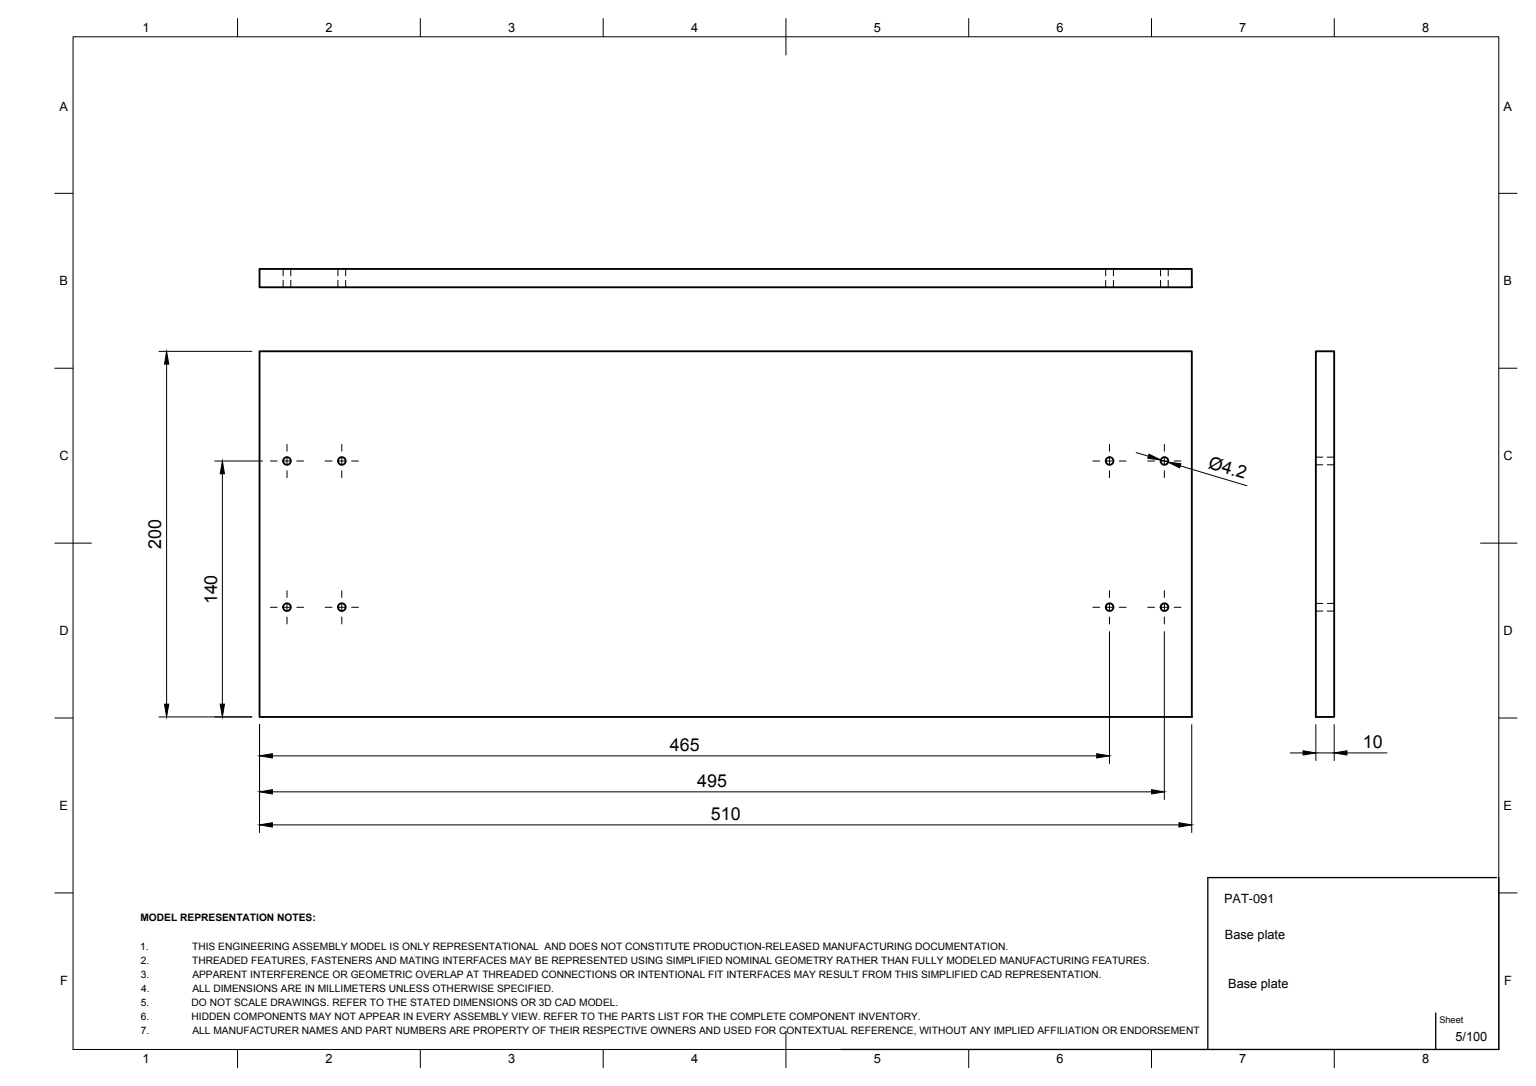
ISO-10303-21;
HEADER;
/* Generated by software containing ST-Developer
 * from STEP Tools, Inc. (www.steptools.com) 
 */

FILE_DESCRIPTION(
/* description */ ('PAT-091'),
/* implementation_level */ '2;1');

FILE_NAME(
/* name */ 'Base plate.step',
/* time_stamp */ '2026-10-27T15:34:44-07:00',
/* author */ (''),
/* organization */ (''),
/* preprocessor_version */ 'ST-DEVELOPER v20.2',
/* originating_system */ 'Autodesk Translation Framework v15.17.0.0',
/* authorisation */ '');

FILE_SCHEMA (('AUTOMOTIVE_DESIGN { 1 0 10303 214 3 1 1 }'));
ENDSEC;

DATA;
#10=MECHANICAL_DESIGN_GEOMETRIC_PRESENTATION_REPRESENTATION('',(#971),#25100);
#751=SHAPE_REPRESENTATION_RELATIONSHIP('SRR','None',#25512,#861);
#861=ADVANCED_BREP_SHAPE_REPRESENTATION('',(#1095),#24982);
#971=STYLED_ITEM('',(#26170),#1095);
#1095=MANIFOLD_SOLID_BREP('Body1',#13248);
#1215=FACE_BOUND('',#2894,.T.);
#1216=FACE_BOUND('',#2895,.T.);
#1217=FACE_BOUND('',#2896,.T.);
#1218=FACE_BOUND('',#2897,.T.);
#1219=FACE_BOUND('',#2898,.T.);
#1220=FACE_BOUND('',#2899,.T.);
#1221=FACE_BOUND('',#2900,.T.);
#1222=FACE_BOUND('',#2901,.T.);
#1223=FACE_BOUND('',#2903,.T.);
#1224=FACE_BOUND('',#2904,.T.);
#1225=FACE_BOUND('',#2905,.T.);
#1226=FACE_BOUND('',#2906,.T.);
#1227=FACE_BOUND('',#2907,.T.);
#1228=FACE_BOUND('',#2908,.T.);
#1229=FACE_BOUND('',#2909,.T.);
#1230=FACE_BOUND('',#2910,.T.);
#1640=PLANE('',#14612);
#1641=PLANE('',#14613);
#1642=PLANE('',#14614);
#1643=PLANE('',#14615);
#1644=PLANE('',#14616);
#1645=PLANE('',#14617);
#2063=FACE_OUTER_BOUND('',#2881,.T.);
#2064=FACE_OUTER_BOUND('',#2882,.T.);
#2065=FACE_OUTER_BOUND('',#2883,.T.);
#2066=FACE_OUTER_BOUND('',#2884,.T.);
#2067=FACE_OUTER_BOUND('',#2885,.T.);
#2068=FACE_OUTER_BOUND('',#2886,.T.);
#2069=FACE_OUTER_BOUND('',#2887,.T.);
#2070=FACE_OUTER_BOUND('',#2888,.T.);
#2071=FACE_OUTER_BOUND('',#2889,.T.);
#2072=FACE_OUTER_BOUND('',#2890,.T.);
#2073=FACE_OUTER_BOUND('',#2891,.T.);
#2074=FACE_OUTER_BOUND('',#2892,.T.);
#2075=FACE_OUTER_BOUND('',#2893,.T.);
#2076=FACE_OUTER_BOUND('',#2902,.T.);
#2881=EDGE_LOOP('',(#8972,#8973,#8974,#8975));
#2882=EDGE_LOOP('',(#8976,#8977,#8978,#8979));
#2883=EDGE_LOOP('',(#8980,#8981,#8982,#8983));
#2884=EDGE_LOOP('',(#8984,#8985,#8986,#8987));
#2885=EDGE_LOOP('',(#8988,#8989,#8990,#8991));
#2886=EDGE_LOOP('',(#8992,#8993,#8994,#8995));
#2887=EDGE_LOOP('',(#8996,#8997,#8998,#8999));
#2888=EDGE_LOOP('',(#9000,#9001,#9002,#9003));
#2889=EDGE_LOOP('',(#9004,#9005,#9006,#9007));
#2890=EDGE_LOOP('',(#9008,#9009,#9010,#9011));
#2891=EDGE_LOOP('',(#9012,#9013,#9014,#9015));
#2892=EDGE_LOOP('',(#9016,#9017,#9018,#9019));
#2893=EDGE_LOOP('',(#9020,#9021,#9022,#9023));
#2894=EDGE_LOOP('',(#9024));
#2895=EDGE_LOOP('',(#9025));
#2896=EDGE_LOOP('',(#9026));
#2897=EDGE_LOOP('',(#9027));
#2898=EDGE_LOOP('',(#9028));
#2899=EDGE_LOOP('',(#9029));
#2900=EDGE_LOOP('',(#9030));
#2901=EDGE_LOOP('',(#9031));
#2902=EDGE_LOOP('',(#9032,#9033,#9034,#9035));
#2903=EDGE_LOOP('',(#9036));
#2904=EDGE_LOOP('',(#9037));
#2905=EDGE_LOOP('',(#9038));
#2906=EDGE_LOOP('',(#9039));
#2907=EDGE_LOOP('',(#9040));
#2908=EDGE_LOOP('',(#9041));
#2909=EDGE_LOOP('',(#9042));
#2910=EDGE_LOOP('',(#9043));
#4124=LINE('',#20981,#4864);
#4125=LINE('',#20987,#4865);
#4126=LINE('',#20993,#4866);
#4127=LINE('',#20999,#4867);
#4128=LINE('',#21005,#4868);
#4129=LINE('',#21011,#4869);
#4130=LINE('',#21017,#4870);
#4131=LINE('',#21023,#4871);
#4132=LINE('',#21028,#4872);
#4133=LINE('',#21030,#4873);
#4134=LINE('',#21032,#4874);
#4135=LINE('',#21033,#4875);
#4136=LINE('',#21036,#4876);
#4137=LINE('',#21038,#4877);
#4138=LINE('',#21039,#4878);
#4139=LINE('',#21042,#4879);
#4140=LINE('',#21044,#4880);
#4141=LINE('',#21045,#4881);
#4142=LINE('',#21047,#4882);
#4143=LINE('',#21048,#4883);
#4864=VECTOR('',#16478,0.210000000000001);
#4865=VECTOR('',#16485,0.210000000000001);
#4866=VECTOR('',#16492,0.210000000000001);
#4867=VECTOR('',#16499,0.210000000000001);
#4868=VECTOR('',#16506,0.21);
#4869=VECTOR('',#16513,0.21);
#4870=VECTOR('',#16520,0.21);
#4871=VECTOR('',#16527,0.21);
#4872=VECTOR('',#16532,1.);
#4873=VECTOR('',#16533,1.);
#4874=VECTOR('',#16534,1.);
#4875=VECTOR('',#16535,1.);
#4876=VECTOR('',#16538,1.);
#4877=VECTOR('',#16539,1.);
#4878=VECTOR('',#16540,1.);
#4879=VECTOR('',#16543,1.);
#4880=VECTOR('',#16544,1.);
#4881=VECTOR('',#16545,1.);
#4882=VECTOR('',#16548,1.);
#4883=VECTOR('',#16549,1.);
#5604=CIRCLE('',#14589,0.210000000000001);
#5605=CIRCLE('',#14590,0.210000000000001);
#5606=CIRCLE('',#14592,0.210000000000001);
#5607=CIRCLE('',#14593,0.210000000000001);
#5608=CIRCLE('',#14595,0.210000000000001);
#5609=CIRCLE('',#14596,0.210000000000001);
#5610=CIRCLE('',#14598,0.210000000000001);
#5611=CIRCLE('',#14599,0.210000000000001);
#5612=CIRCLE('',#14601,0.21);
#5613=CIRCLE('',#14602,0.21);
#5614=CIRCLE('',#14604,0.21);
#5615=CIRCLE('',#14605,0.21);
#5616=CIRCLE('',#14607,0.21);
#5617=CIRCLE('',#14608,0.21);
#5618=CIRCLE('',#14610,0.21);
#5619=CIRCLE('',#14611,0.21);
#6383=VERTEX_POINT('',#20978);
#6384=VERTEX_POINT('',#20980);
#6385=VERTEX_POINT('',#20984);
#6386=VERTEX_POINT('',#20986);
#6387=VERTEX_POINT('',#20990);
#6388=VERTEX_POINT('',#20992);
#6389=VERTEX_POINT('',#20996);
#6390=VERTEX_POINT('',#20998);
#6391=VERTEX_POINT('',#21002);
#6392=VERTEX_POINT('',#21004);
#6393=VERTEX_POINT('',#21008);
#6394=VERTEX_POINT('',#21010);
#6395=VERTEX_POINT('',#21014);
#6396=VERTEX_POINT('',#21016);
#6397=VERTEX_POINT('',#21020);
#6398=VERTEX_POINT('',#21022);
#6399=VERTEX_POINT('',#21026);
#6400=VERTEX_POINT('',#21027);
#6401=VERTEX_POINT('',#21029);
#6402=VERTEX_POINT('',#21031);
#6403=VERTEX_POINT('',#21035);
#6404=VERTEX_POINT('',#21037);
#6405=VERTEX_POINT('',#21041);
#6406=VERTEX_POINT('',#21043);
#7421=EDGE_CURVE('',#6383,#6383,#5604,.T.);
#7422=EDGE_CURVE('',#6383,#6384,#4124,.T.);
#7423=EDGE_CURVE('',#6384,#6384,#5605,.T.);
#7424=EDGE_CURVE('',#6385,#6385,#5606,.T.);
#7425=EDGE_CURVE('',#6385,#6386,#4125,.T.);
#7426=EDGE_CURVE('',#6386,#6386,#5607,.T.);
#7427=EDGE_CURVE('',#6387,#6387,#5608,.T.);
#7428=EDGE_CURVE('',#6387,#6388,#4126,.T.);
#7429=EDGE_CURVE('',#6388,#6388,#5609,.T.);
#7430=EDGE_CURVE('',#6389,#6389,#5610,.T.);
#7431=EDGE_CURVE('',#6389,#6390,#4127,.T.);
#7432=EDGE_CURVE('',#6390,#6390,#5611,.T.);
#7433=EDGE_CURVE('',#6391,#6391,#5612,.T.);
#7434=EDGE_CURVE('',#6391,#6392,#4128,.T.);
#7435=EDGE_CURVE('',#6392,#6392,#5613,.T.);
#7436=EDGE_CURVE('',#6393,#6393,#5614,.T.);
#7437=EDGE_CURVE('',#6393,#6394,#4129,.T.);
#7438=EDGE_CURVE('',#6394,#6394,#5615,.T.);
#7439=EDGE_CURVE('',#6395,#6395,#5616,.T.);
#7440=EDGE_CURVE('',#6395,#6396,#4130,.T.);
#7441=EDGE_CURVE('',#6396,#6396,#5617,.T.);
#7442=EDGE_CURVE('',#6397,#6397,#5618,.T.);
#7443=EDGE_CURVE('',#6397,#6398,#4131,.T.);
#7444=EDGE_CURVE('',#6398,#6398,#5619,.T.);
#7445=EDGE_CURVE('',#6399,#6400,#4132,.T.);
#7446=EDGE_CURVE('',#6400,#6401,#4133,.T.);
#7447=EDGE_CURVE('',#6402,#6401,#4134,.T.);
#7448=EDGE_CURVE('',#6399,#6402,#4135,.T.);
#7449=EDGE_CURVE('',#6403,#6399,#4136,.T.);
#7450=EDGE_CURVE('',#6404,#6402,#4137,.T.);
#7451=EDGE_CURVE('',#6403,#6404,#4138,.T.);
#7452=EDGE_CURVE('',#6405,#6403,#4139,.T.);
#7453=EDGE_CURVE('',#6406,#6404,#4140,.T.);
#7454=EDGE_CURVE('',#6405,#6406,#4141,.T.);
#7455=EDGE_CURVE('',#6400,#6405,#4142,.T.);
#7456=EDGE_CURVE('',#6401,#6406,#4143,.T.);
#8972=ORIENTED_EDGE('',*,*,#7421,.F.);
#8973=ORIENTED_EDGE('',*,*,#7422,.T.);
#8974=ORIENTED_EDGE('',*,*,#7423,.F.);
#8975=ORIENTED_EDGE('',*,*,#7422,.F.);
#8976=ORIENTED_EDGE('',*,*,#7424,.F.);
#8977=ORIENTED_EDGE('',*,*,#7425,.T.);
#8978=ORIENTED_EDGE('',*,*,#7426,.F.);
#8979=ORIENTED_EDGE('',*,*,#7425,.F.);
#8980=ORIENTED_EDGE('',*,*,#7427,.F.);
#8981=ORIENTED_EDGE('',*,*,#7428,.T.);
#8982=ORIENTED_EDGE('',*,*,#7429,.F.);
#8983=ORIENTED_EDGE('',*,*,#7428,.F.);
#8984=ORIENTED_EDGE('',*,*,#7430,.F.);
#8985=ORIENTED_EDGE('',*,*,#7431,.T.);
#8986=ORIENTED_EDGE('',*,*,#7432,.F.);
#8987=ORIENTED_EDGE('',*,*,#7431,.F.);
#8988=ORIENTED_EDGE('',*,*,#7433,.F.);
#8989=ORIENTED_EDGE('',*,*,#7434,.T.);
#8990=ORIENTED_EDGE('',*,*,#7435,.F.);
#8991=ORIENTED_EDGE('',*,*,#7434,.F.);
#8992=ORIENTED_EDGE('',*,*,#7436,.F.);
#8993=ORIENTED_EDGE('',*,*,#7437,.T.);
#8994=ORIENTED_EDGE('',*,*,#7438,.F.);
#8995=ORIENTED_EDGE('',*,*,#7437,.F.);
#8996=ORIENTED_EDGE('',*,*,#7439,.F.);
#8997=ORIENTED_EDGE('',*,*,#7440,.T.);
#8998=ORIENTED_EDGE('',*,*,#7441,.F.);
#8999=ORIENTED_EDGE('',*,*,#7440,.F.);
#9000=ORIENTED_EDGE('',*,*,#7442,.F.);
#9001=ORIENTED_EDGE('',*,*,#7443,.T.);
#9002=ORIENTED_EDGE('',*,*,#7444,.F.);
#9003=ORIENTED_EDGE('',*,*,#7443,.F.);
#9004=ORIENTED_EDGE('',*,*,#7445,.T.);
#9005=ORIENTED_EDGE('',*,*,#7446,.T.);
#9006=ORIENTED_EDGE('',*,*,#7447,.F.);
#9007=ORIENTED_EDGE('',*,*,#7448,.F.);
#9008=ORIENTED_EDGE('',*,*,#7449,.T.);
#9009=ORIENTED_EDGE('',*,*,#7448,.T.);
#9010=ORIENTED_EDGE('',*,*,#7450,.F.);
#9011=ORIENTED_EDGE('',*,*,#7451,.F.);
#9012=ORIENTED_EDGE('',*,*,#7452,.T.);
#9013=ORIENTED_EDGE('',*,*,#7451,.T.);
#9014=ORIENTED_EDGE('',*,*,#7453,.F.);
#9015=ORIENTED_EDGE('',*,*,#7454,.F.);
#9016=ORIENTED_EDGE('',*,*,#7455,.T.);
#9017=ORIENTED_EDGE('',*,*,#7454,.T.);
#9018=ORIENTED_EDGE('',*,*,#7456,.F.);
#9019=ORIENTED_EDGE('',*,*,#7446,.F.);
#9020=ORIENTED_EDGE('',*,*,#7456,.T.);
#9021=ORIENTED_EDGE('',*,*,#7453,.T.);
#9022=ORIENTED_EDGE('',*,*,#7450,.T.);
#9023=ORIENTED_EDGE('',*,*,#7447,.T.);
#9024=ORIENTED_EDGE('',*,*,#7444,.T.);
#9025=ORIENTED_EDGE('',*,*,#7441,.T.);
#9026=ORIENTED_EDGE('',*,*,#7438,.T.);
#9027=ORIENTED_EDGE('',*,*,#7435,.T.);
#9028=ORIENTED_EDGE('',*,*,#7432,.T.);
#9029=ORIENTED_EDGE('',*,*,#7429,.T.);
#9030=ORIENTED_EDGE('',*,*,#7426,.T.);
#9031=ORIENTED_EDGE('',*,*,#7423,.T.);
#9032=ORIENTED_EDGE('',*,*,#7455,.F.);
#9033=ORIENTED_EDGE('',*,*,#7445,.F.);
#9034=ORIENTED_EDGE('',*,*,#7449,.F.);
#9035=ORIENTED_EDGE('',*,*,#7452,.F.);
#9036=ORIENTED_EDGE('',*,*,#7442,.T.);
#9037=ORIENTED_EDGE('',*,*,#7439,.T.);
#9038=ORIENTED_EDGE('',*,*,#7436,.T.);
#9039=ORIENTED_EDGE('',*,*,#7433,.T.);
#9040=ORIENTED_EDGE('',*,*,#7430,.T.);
#9041=ORIENTED_EDGE('',*,*,#7427,.T.);
#9042=ORIENTED_EDGE('',*,*,#7424,.T.);
#9043=ORIENTED_EDGE('',*,*,#7421,.T.);
#12074=CYLINDRICAL_SURFACE('',#14588,0.210000000000001);
#12075=CYLINDRICAL_SURFACE('',#14591,0.210000000000001);
#12076=CYLINDRICAL_SURFACE('',#14594,0.210000000000001);
#12077=CYLINDRICAL_SURFACE('',#14597,0.210000000000001);
#12078=CYLINDRICAL_SURFACE('',#14600,0.21);
#12079=CYLINDRICAL_SURFACE('',#14603,0.21);
#12080=CYLINDRICAL_SURFACE('',#14606,0.21);
#12081=CYLINDRICAL_SURFACE('',#14609,0.21);
#12430=ADVANCED_FACE('',(#2063),#12074,.F.);
#12431=ADVANCED_FACE('',(#2064),#12075,.F.);
#12432=ADVANCED_FACE('',(#2065),#12076,.F.);
#12433=ADVANCED_FACE('',(#2066),#12077,.F.);
#12434=ADVANCED_FACE('',(#2067),#12078,.F.);
#12435=ADVANCED_FACE('',(#2068),#12079,.F.);
#12436=ADVANCED_FACE('',(#2069),#12080,.F.);
#12437=ADVANCED_FACE('',(#2070),#12081,.F.);
#12438=ADVANCED_FACE('',(#2071),#1640,.T.);
#12439=ADVANCED_FACE('',(#2072),#1641,.T.);
#12440=ADVANCED_FACE('',(#2073),#1642,.T.);
#12441=ADVANCED_FACE('',(#2074),#1643,.T.);
#12442=ADVANCED_FACE('',(#2075,#1215,#1216,#1217,#1218,#1219,#1220,#1221,
#1222),#1644,.T.);
#12443=ADVANCED_FACE('',(#2076,#1223,#1224,#1225,#1226,#1227,#1228,#1229,
#1230),#1645,.F.);
#13248=CLOSED_SHELL('',(#12430,#12431,#12432,#12433,#12434,#12435,#12436,
#12437,#12438,#12439,#12440,#12441,#12442,#12443));
#14587=AXIS2_PLACEMENT_3D('',#20976,#16472,#16473);
#14588=AXIS2_PLACEMENT_3D('',#20977,#16474,#16475);
#14589=AXIS2_PLACEMENT_3D('',#20979,#16476,#16477);
#14590=AXIS2_PLACEMENT_3D('',#20982,#16479,#16480);
#14591=AXIS2_PLACEMENT_3D('',#20983,#16481,#16482);
#14592=AXIS2_PLACEMENT_3D('',#20985,#16483,#16484);
#14593=AXIS2_PLACEMENT_3D('',#20988,#16486,#16487);
#14594=AXIS2_PLACEMENT_3D('',#20989,#16488,#16489);
#14595=AXIS2_PLACEMENT_3D('',#20991,#16490,#16491);
#14596=AXIS2_PLACEMENT_3D('',#20994,#16493,#16494);
#14597=AXIS2_PLACEMENT_3D('',#20995,#16495,#16496);
#14598=AXIS2_PLACEMENT_3D('',#20997,#16497,#16498);
#14599=AXIS2_PLACEMENT_3D('',#21000,#16500,#16501);
#14600=AXIS2_PLACEMENT_3D('',#21001,#16502,#16503);
#14601=AXIS2_PLACEMENT_3D('',#21003,#16504,#16505);
#14602=AXIS2_PLACEMENT_3D('',#21006,#16507,#16508);
#14603=AXIS2_PLACEMENT_3D('',#21007,#16509,#16510);
#14604=AXIS2_PLACEMENT_3D('',#21009,#16511,#16512);
#14605=AXIS2_PLACEMENT_3D('',#21012,#16514,#16515);
#14606=AXIS2_PLACEMENT_3D('',#21013,#16516,#16517);
#14607=AXIS2_PLACEMENT_3D('',#21015,#16518,#16519);
#14608=AXIS2_PLACEMENT_3D('',#21018,#16521,#16522);
#14609=AXIS2_PLACEMENT_3D('',#21019,#16523,#16524);
#14610=AXIS2_PLACEMENT_3D('',#21021,#16525,#16526);
#14611=AXIS2_PLACEMENT_3D('',#21024,#16528,#16529);
#14612=AXIS2_PLACEMENT_3D('',#21025,#16530,#16531);
#14613=AXIS2_PLACEMENT_3D('',#21034,#16536,#16537);
#14614=AXIS2_PLACEMENT_3D('',#21040,#16541,#16542);
#14615=AXIS2_PLACEMENT_3D('',#21046,#16546,#16547);
#14616=AXIS2_PLACEMENT_3D('',#21049,#16550,#16551);
#14617=AXIS2_PLACEMENT_3D('',#21050,#16552,#16553);
#16472=DIRECTION('axis',(0.,0.,1.));
#16473=DIRECTION('refdir',(1.,0.,0.));
#16474=DIRECTION('center_axis',(0.,0.,1.));
#16475=DIRECTION('ref_axis',(1.,0.,0.));
#16476=DIRECTION('center_axis',(0.,0.,1.));
#16477=DIRECTION('ref_axis',(1.,0.,0.));
#16478=DIRECTION('',(0.,0.,1.));
#16479=DIRECTION('center_axis',(0.,0.,-1.));
#16480=DIRECTION('ref_axis',(1.,0.,0.));
#16481=DIRECTION('center_axis',(0.,0.,1.));
#16482=DIRECTION('ref_axis',(1.,0.,0.));
#16483=DIRECTION('center_axis',(0.,0.,1.));
#16484=DIRECTION('ref_axis',(1.,0.,0.));
#16485=DIRECTION('',(0.,0.,1.));
#16486=DIRECTION('center_axis',(0.,0.,-1.));
#16487=DIRECTION('ref_axis',(1.,0.,0.));
#16488=DIRECTION('center_axis',(0.,0.,1.));
#16489=DIRECTION('ref_axis',(1.,0.,0.));
#16490=DIRECTION('center_axis',(0.,0.,1.));
#16491=DIRECTION('ref_axis',(1.,0.,0.));
#16492=DIRECTION('',(0.,0.,1.));
#16493=DIRECTION('center_axis',(0.,0.,-1.));
#16494=DIRECTION('ref_axis',(1.,0.,0.));
#16495=DIRECTION('center_axis',(0.,0.,1.));
#16496=DIRECTION('ref_axis',(1.,0.,0.));
#16497=DIRECTION('center_axis',(0.,0.,1.));
#16498=DIRECTION('ref_axis',(1.,0.,0.));
#16499=DIRECTION('',(0.,0.,1.));
#16500=DIRECTION('center_axis',(0.,0.,-1.));
#16501=DIRECTION('ref_axis',(1.,0.,0.));
#16502=DIRECTION('center_axis',(0.,0.,1.));
#16503=DIRECTION('ref_axis',(1.,0.,0.));
#16504=DIRECTION('center_axis',(0.,0.,1.));
#16505=DIRECTION('ref_axis',(1.,0.,0.));
#16506=DIRECTION('',(0.,0.,1.));
#16507=DIRECTION('center_axis',(0.,0.,-1.));
#16508=DIRECTION('ref_axis',(1.,0.,0.));
#16509=DIRECTION('center_axis',(0.,0.,1.));
#16510=DIRECTION('ref_axis',(1.,0.,0.));
#16511=DIRECTION('center_axis',(0.,0.,1.));
#16512=DIRECTION('ref_axis',(1.,0.,0.));
#16513=DIRECTION('',(0.,0.,1.));
#16514=DIRECTION('center_axis',(0.,0.,-1.));
#16515=DIRECTION('ref_axis',(1.,0.,0.));
#16516=DIRECTION('center_axis',(0.,0.,1.));
#16517=DIRECTION('ref_axis',(1.,0.,0.));
#16518=DIRECTION('center_axis',(0.,0.,1.));
#16519=DIRECTION('ref_axis',(1.,0.,0.));
#16520=DIRECTION('',(0.,0.,1.));
#16521=DIRECTION('center_axis',(0.,0.,-1.));
#16522=DIRECTION('ref_axis',(1.,0.,0.));
#16523=DIRECTION('center_axis',(0.,0.,1.));
#16524=DIRECTION('ref_axis',(1.,0.,0.));
#16525=DIRECTION('center_axis',(0.,0.,1.));
#16526=DIRECTION('ref_axis',(1.,0.,0.));
#16527=DIRECTION('',(0.,0.,1.));
#16528=DIRECTION('center_axis',(0.,0.,-1.));
#16529=DIRECTION('ref_axis',(1.,0.,0.));
#16530=DIRECTION('center_axis',(0.,1.,0.));
#16531=DIRECTION('ref_axis',(-1.,0.,0.));
#16532=DIRECTION('',(-1.,0.,0.));
#16533=DIRECTION('',(0.,0.,1.));
#16534=DIRECTION('',(-1.,0.,0.));
#16535=DIRECTION('',(0.,0.,1.));
#16536=DIRECTION('center_axis',(1.,0.,0.));
#16537=DIRECTION('ref_axis',(0.,1.,0.));
#16538=DIRECTION('',(0.,1.,0.));
#16539=DIRECTION('',(0.,1.,0.));
#16540=DIRECTION('',(0.,0.,1.));
#16541=DIRECTION('center_axis',(0.,-1.,0.));
#16542=DIRECTION('ref_axis',(1.,0.,0.));
#16543=DIRECTION('',(1.,0.,0.));
#16544=DIRECTION('',(1.,0.,0.));
#16545=DIRECTION('',(0.,0.,1.));
#16546=DIRECTION('center_axis',(-1.,0.,0.));
#16547=DIRECTION('ref_axis',(0.,-1.,0.));
#16548=DIRECTION('',(0.,-1.,0.));
#16549=DIRECTION('',(0.,-1.,0.));
#16550=DIRECTION('center_axis',(0.,0.,1.));
#16551=DIRECTION('ref_axis',(1.,0.,0.));
#16552=DIRECTION('center_axis',(0.,0.,1.));
#16553=DIRECTION('ref_axis',(1.,0.,0.));
#20976=CARTESIAN_POINT('',(0.,0.,0.));
#20977=CARTESIAN_POINT('Origin',(46.5,-4.,-0.1));
#20978=CARTESIAN_POINT('',(46.29,-4.,0.));
#20979=CARTESIAN_POINT('Origin',(46.5,-4.,0.));
#20980=CARTESIAN_POINT('',(46.29,-4.,1.));
#20981=CARTESIAN_POINT('',(46.29,-4.,-0.1));
#20982=CARTESIAN_POINT('Origin',(46.5,-4.,1.));
#20983=CARTESIAN_POINT('Origin',(43.5,4.,-0.1));
#20984=CARTESIAN_POINT('',(43.29,4.,0.));
#20985=CARTESIAN_POINT('Origin',(43.5,4.,0.));
#20986=CARTESIAN_POINT('',(43.29,4.,1.));
#20987=CARTESIAN_POINT('',(43.29,4.,-0.1));
#20988=CARTESIAN_POINT('Origin',(43.5,4.,1.));
#20989=CARTESIAN_POINT('Origin',(43.5,-4.,-0.1));
#20990=CARTESIAN_POINT('',(43.29,-4.,0.));
#20991=CARTESIAN_POINT('Origin',(43.5,-4.,0.));
#20992=CARTESIAN_POINT('',(43.29,-4.,1.));
#20993=CARTESIAN_POINT('',(43.29,-4.,-0.1));
#20994=CARTESIAN_POINT('Origin',(43.5,-4.,1.));
#20995=CARTESIAN_POINT('Origin',(46.5,4.,-0.1));
#20996=CARTESIAN_POINT('',(46.29,4.,0.));
#20997=CARTESIAN_POINT('Origin',(46.5,4.,0.));
#20998=CARTESIAN_POINT('',(46.29,4.,1.));
#20999=CARTESIAN_POINT('',(46.29,4.,-0.1));
#21000=CARTESIAN_POINT('Origin',(46.5,4.,1.));
#21001=CARTESIAN_POINT('Origin',(1.5,-4.,-0.1));
#21002=CARTESIAN_POINT('',(1.29,-4.,0.));
#21003=CARTESIAN_POINT('Origin',(1.5,-4.,0.));
#21004=CARTESIAN_POINT('',(1.29,-4.,1.));
#21005=CARTESIAN_POINT('',(1.29,-4.,-0.1));
#21006=CARTESIAN_POINT('Origin',(1.5,-4.,1.));
#21007=CARTESIAN_POINT('Origin',(-1.5,4.,-0.1));
#21008=CARTESIAN_POINT('',(-1.71,4.,0.));
#21009=CARTESIAN_POINT('Origin',(-1.5,4.,0.));
#21010=CARTESIAN_POINT('',(-1.71,4.,1.));
#21011=CARTESIAN_POINT('',(-1.71,4.,-0.1));
#21012=CARTESIAN_POINT('Origin',(-1.5,4.,1.));
#21013=CARTESIAN_POINT('Origin',(-1.5,-4.,-0.1));
#21014=CARTESIAN_POINT('',(-1.71,-4.,0.));
#21015=CARTESIAN_POINT('Origin',(-1.5,-4.,0.));
#21016=CARTESIAN_POINT('',(-1.71,-4.,1.));
#21017=CARTESIAN_POINT('',(-1.71,-4.,-0.1));
#21018=CARTESIAN_POINT('Origin',(-1.5,-4.,1.));
#21019=CARTESIAN_POINT('Origin',(1.5,4.,-0.1));
#21020=CARTESIAN_POINT('',(1.29,4.,0.));
#21021=CARTESIAN_POINT('Origin',(1.5,4.,0.));
#21022=CARTESIAN_POINT('',(1.29,4.,1.));
#21023=CARTESIAN_POINT('',(1.29,4.,-0.1));
#21024=CARTESIAN_POINT('Origin',(1.5,4.,1.));
#21025=CARTESIAN_POINT('Origin',(48.,10.,0.));
#21026=CARTESIAN_POINT('',(48.,10.,0.));
#21027=CARTESIAN_POINT('',(-3.,10.,0.));
#21028=CARTESIAN_POINT('',(48.,10.,0.));
#21029=CARTESIAN_POINT('',(-3.,10.,1.));
#21030=CARTESIAN_POINT('',(-3.,10.,0.));
#21031=CARTESIAN_POINT('',(48.,10.,1.));
#21032=CARTESIAN_POINT('',(48.,10.,1.));
#21033=CARTESIAN_POINT('',(48.,10.,0.));
#21034=CARTESIAN_POINT('Origin',(48.,-10.,0.));
#21035=CARTESIAN_POINT('',(48.,-10.,0.));
#21036=CARTESIAN_POINT('',(48.,-10.,0.));
#21037=CARTESIAN_POINT('',(48.,-10.,1.));
#21038=CARTESIAN_POINT('',(48.,-10.,1.));
#21039=CARTESIAN_POINT('',(48.,-10.,0.));
#21040=CARTESIAN_POINT('Origin',(-3.,-10.,0.));
#21041=CARTESIAN_POINT('',(-3.,-10.,0.));
#21042=CARTESIAN_POINT('',(-3.,-10.,0.));
#21043=CARTESIAN_POINT('',(-3.,-10.,1.));
#21044=CARTESIAN_POINT('',(-3.,-10.,1.));
#21045=CARTESIAN_POINT('',(-3.,-10.,0.));
#21046=CARTESIAN_POINT('Origin',(-3.,10.,0.));
#21047=CARTESIAN_POINT('',(-3.,10.,0.));
#21048=CARTESIAN_POINT('',(-3.,10.,1.));
#21049=CARTESIAN_POINT('Origin',(22.5,0.,1.));
#21050=CARTESIAN_POINT('Origin',(22.5,0.,0.));
#24861=UNCERTAINTY_MEASURE_WITH_UNIT(LENGTH_MEASURE(0.001),#25101,
'DISTANCE_ACCURACY_VALUE',
'Maximum model space distance between geometric entities at asserted c
onnectivities');
#24979=UNCERTAINTY_MEASURE_WITH_UNIT(LENGTH_MEASURE(0.001),#25101,
'DISTANCE_ACCURACY_VALUE',
'Maximum model space distance between geometric entities at asserted c
onnectivities');
#24982=(
GEOMETRIC_REPRESENTATION_CONTEXT(3)
GLOBAL_UNCERTAINTY_ASSIGNED_CONTEXT((#24861))
GLOBAL_UNIT_ASSIGNED_CONTEXT((#25101,#25103,#25104))
REPRESENTATION_CONTEXT('','3D')
);
#25100=(
GEOMETRIC_REPRESENTATION_CONTEXT(3)
GLOBAL_UNCERTAINTY_ASSIGNED_CONTEXT((#24979))
GLOBAL_UNIT_ASSIGNED_CONTEXT((#25101,#25103,#25104))
REPRESENTATION_CONTEXT('','3D')
);
#25101=(
LENGTH_UNIT()
NAMED_UNIT(*)
SI_UNIT(.CENTI.,.METRE.)
);
#25103=(
NAMED_UNIT(*)
PLANE_ANGLE_UNIT()
SI_UNIT($,.RADIAN.)
);
#25104=(
NAMED_UNIT(*)
SI_UNIT($,.STERADIAN.)
SOLID_ANGLE_UNIT()
);
#25107=SHAPE_DEFINITION_REPRESENTATION(#25227,#25512);
#25227=PRODUCT_DEFINITION_SHAPE('',$,#25633);
#25512=SHAPE_REPRESENTATION('',(#14587),#24982);
#25630=PRODUCT_DEFINITION_CONTEXT('part definition',#25992,'design');
#25633=PRODUCT_DEFINITION('Base plate','Base plate',#25753,#25630);
#25753=PRODUCT_DEFINITION_FORMATION('',$,#25996);
#25992=APPLICATION_CONTEXT(
'Core Data for Automotive Mechanical Design Process');
#25993=PRODUCT_CONTEXT('part definition',#25992,'mechanical');
#25996=PRODUCT('Base plate','Base plate','Base plate',(#25993));
#26164=COLOUR_RGB('Dark Blue',0.08,0.2,0.34);
#26165=FILL_AREA_STYLE_COLOUR('',#26164);
#26166=FILL_AREA_STYLE('',(#26165));
#26167=SURFACE_STYLE_FILL_AREA(#26166);
#26168=SURFACE_SIDE_STYLE('',(#26167));
#26169=SURFACE_STYLE_USAGE(.BOTH.,#26168);
#26170=PRESENTATION_STYLE_ASSIGNMENT((#26169));
ENDSEC;
END-ISO-10303-21;
